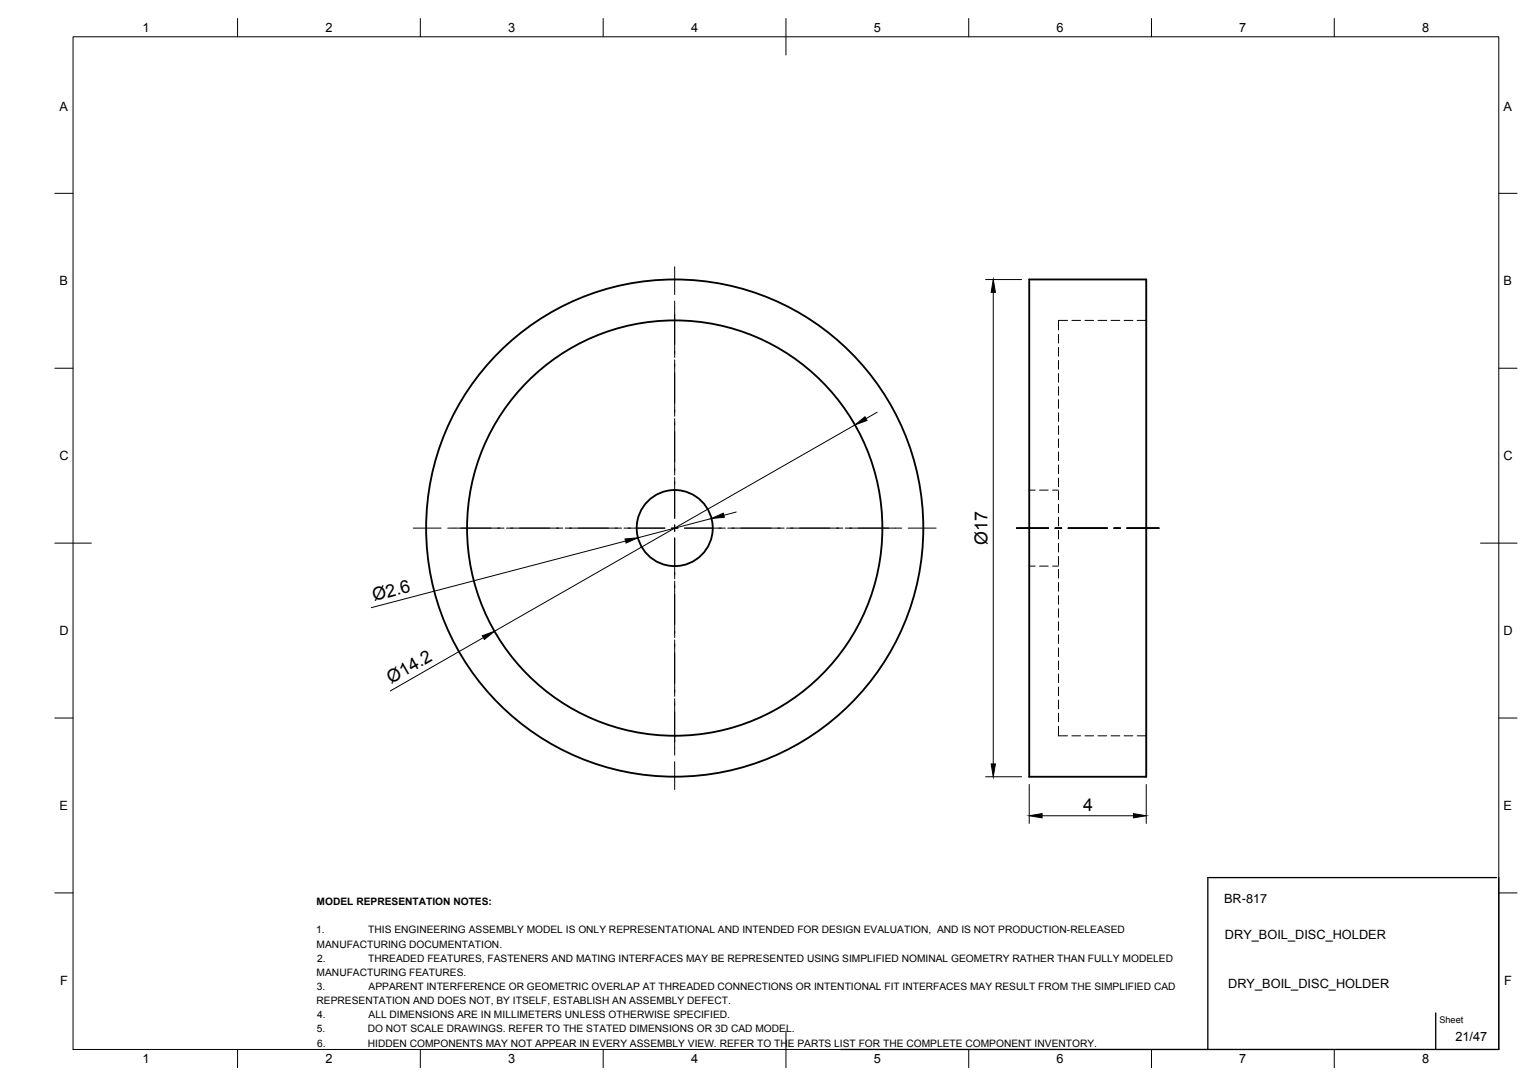
ISO-10303-21;
HEADER;
FILE_DESCRIPTION((''),'2;1');
FILE_NAME('DRY_BOIL_DISC_HOLDER.step','2026-10-01T22:07:29-07:00',(''),(''),'','','');
FILE_SCHEMA (('AUTOMOTIVE_DESIGN { 1 0 10303 214 3 1 1 }'));
ENDSEC;
DATA;
#10=MECHANICAL_DESIGN_GEOMETRIC_PRESENTATION_REPRESENTATION('',(#555),#15484);
#485=SHAPE_REPRESENTATION_RELATIONSHIP('SRR','None',#15634,#520) ;
#520=ADVANCED_BREP_SHAPE_REPRESENTATION('',(#596),#15458) ;
#555=STYLED_ITEM('',(#15834),#596) ;
#596=MANIFOLD_SOLID_BREP('DRY_BOIL_DISC_HOLDER',#8266) ;
#677=CYLINDRICAL_SURFACE('',#8977,0.13) ;
#678=CYLINDRICAL_SURFACE('',#8980,0.71) ;
#679=CYLINDRICAL_SURFACE('',#8985,0.85) ;
#863=FACE_BOUND('',#2079,.T.) ;
#864=FACE_BOUND('',#2082,.T.) ;
#865=FACE_BOUND('',#2084,.T.) ;
#997=CIRCLE('',#8978,0.13) ;
#998=CIRCLE('',#8979,0.13) ;
#999=CIRCLE('',#8981,0.71) ;
#1000=CIRCLE('',#8982,0.71) ;
#1001=CIRCLE('',#8984,0.85) ;
#1002=CIRCLE('',#8986,0.85) ;
#1523=FACE_OUTER_BOUND('',#2076,.T.) ;
#1524=FACE_OUTER_BOUND('',#2077,.T.) ;
#1525=FACE_OUTER_BOUND('',#2078,.T.) ;
#1526=FACE_OUTER_BOUND('',#2080,.T.) ;
#1527=FACE_OUTER_BOUND('',#2081,.T.) ;
#1528=FACE_OUTER_BOUND('',#2083,.T.) ;
#2076=EDGE_LOOP('',(#5913,#5914,#5915,#5916)) ;
#2077=EDGE_LOOP('',(#5917,#5918,#5919,#5920)) ;
#2078=EDGE_LOOP('',(#5921)) ;
#2079=EDGE_LOOP('',(#5922)) ;
#2080=EDGE_LOOP('',(#5923,#5924,#5925,#5926)) ;
#2081=EDGE_LOOP('',(#5927)) ;
#2082=EDGE_LOOP('',(#5928)) ;
#2083=EDGE_LOOP('',(#5929)) ;
#2084=EDGE_LOOP('',(#5930)) ;
#2644=LINE('',#13647,#3118) ;
#2645=LINE('',#13653,#3119) ;
#2646=LINE('',#13660,#3120) ;
#3118=VECTOR('',#10723,0.13) ;
#3119=VECTOR('',#10730,0.71) ;
#3120=VECTOR('',#10739,0.85) ;
#3603=VERTEX_POINT('',#13644) ;
#3604=VERTEX_POINT('',#13646) ;
#3605=VERTEX_POINT('',#13650) ;
#3606=VERTEX_POINT('',#13652) ;
#3607=VERTEX_POINT('',#13656) ;
#3608=VERTEX_POINT('',#13659) ;
#4461=EDGE_CURVE('',#3603,#3603,#997,.T.) ;
#4462=EDGE_CURVE('',#3603,#3604,#2644,.T.) ;
#4463=EDGE_CURVE('',#3604,#3604,#998,.T.) ;
#4464=EDGE_CURVE('',#3605,#3605,#999,.T.) ;
#4465=EDGE_CURVE('',#3605,#3606,#2645,.T.) ;
#4466=EDGE_CURVE('',#3606,#3606,#1000,.T.) ;
#4467=EDGE_CURVE('',#3607,#3607,#1001,.T.) ;
#4468=EDGE_CURVE('',#3607,#3608,#2646,.T.) ;
#4469=EDGE_CURVE('',#3608,#3608,#1002,.T.) ;
#5913=ORIENTED_EDGE('',*,*,#4461,.F.) ;
#5914=ORIENTED_EDGE('',*,*,#4462,.T.) ;
#5915=ORIENTED_EDGE('',*,*,#4463,.F.) ;
#5916=ORIENTED_EDGE('',*,*,#4462,.F.) ;
#5917=ORIENTED_EDGE('',*,*,#4464,.F.) ;
#5918=ORIENTED_EDGE('',*,*,#4465,.T.) ;
#5919=ORIENTED_EDGE('',*,*,#4466,.F.) ;
#5920=ORIENTED_EDGE('',*,*,#4465,.F.) ;
#5921=ORIENTED_EDGE('',*,*,#4467,.T.) ;
#5922=ORIENTED_EDGE('',*,*,#4466,.T.) ;
#5923=ORIENTED_EDGE('',*,*,#4467,.F.) ;
#5924=ORIENTED_EDGE('',*,*,#4468,.T.) ;
#5925=ORIENTED_EDGE('',*,*,#4469,.F.) ;
#5926=ORIENTED_EDGE('',*,*,#4468,.F.) ;
#5927=ORIENTED_EDGE('',*,*,#4469,.T.) ;
#5928=ORIENTED_EDGE('',*,*,#4461,.T.) ;
#5929=ORIENTED_EDGE('',*,*,#4464,.T.) ;
#5930=ORIENTED_EDGE('',*,*,#4463,.T.) ;
#7638=PLANE('',#8983) ;
#7639=PLANE('',#8987) ;
#7640=PLANE('',#8988) ;
#7910=ADVANCED_FACE('',(#1523),#677,.F.) ;
#7911=ADVANCED_FACE('',(#1524),#678,.F.) ;
#7912=ADVANCED_FACE('',(#1525,#863),#7638,.T.) ;
#7913=ADVANCED_FACE('',(#1526),#679,.T.) ;
#7914=ADVANCED_FACE('',(#1527,#864),#7639,.T.) ;
#7915=ADVANCED_FACE('',(#1528,#865),#7640,.T.) ;
#8266=CLOSED_SHELL('',(#7910,#7911,#7912,#7913,#7914,#7915)) ;
#8976=AXIS2_PLACEMENT_3D('',#13642,#10717,#10718) ;
#8977=AXIS2_PLACEMENT_3D('',#13643,#10719,#10720) ;
#8978=AXIS2_PLACEMENT_3D('',#13645,#10721,#10722) ;
#8979=AXIS2_PLACEMENT_3D('',#13648,#10724,#10725) ;
#8980=AXIS2_PLACEMENT_3D('',#13649,#10726,#10727) ;
#8981=AXIS2_PLACEMENT_3D('',#13651,#10728,#10729) ;
#8982=AXIS2_PLACEMENT_3D('',#13654,#10731,#10732) ;
#8983=AXIS2_PLACEMENT_3D('',#13655,#10733,#10734) ;
#8984=AXIS2_PLACEMENT_3D('',#13657,#10735,#10736) ;
#8985=AXIS2_PLACEMENT_3D('',#13658,#10737,#10738) ;
#8986=AXIS2_PLACEMENT_3D('',#13661,#10740,#10741) ;
#8987=AXIS2_PLACEMENT_3D('',#13662,#10742,#10743) ;
#8988=AXIS2_PLACEMENT_3D('',#13663,#10744,#10745) ;
#10717=DIRECTION('axis',(0.,0.,1.)) ;
#10718=DIRECTION('refdir',(1.,0.,0.)) ;
#10719=DIRECTION('center_axis',(0.,0.,1.)) ;
#10720=DIRECTION('ref_axis',(1.,0.,0.)) ;
#10721=DIRECTION('center_axis',(0.,0.,1.)) ;
#10722=DIRECTION('ref_axis',(1.,0.,0.)) ;
#10723=DIRECTION('',(0.,0.,1.)) ;
#10724=DIRECTION('center_axis',(0.,0.,-1.)) ;
#10725=DIRECTION('ref_axis',(1.,0.,0.)) ;
#10726=DIRECTION('center_axis',(0.,0.,1.)) ;
#10727=DIRECTION('ref_axis',(1.,0.,0.)) ;
#10728=DIRECTION('center_axis',(0.,0.,1.)) ;
#10729=DIRECTION('ref_axis',(1.,0.,0.)) ;
#10730=DIRECTION('',(0.,0.,1.)) ;
#10731=DIRECTION('center_axis',(0.,0.,-1.)) ;
#10732=DIRECTION('ref_axis',(1.,0.,0.)) ;
#10733=DIRECTION('center_axis',(0.,0.,1.)) ;
#10734=DIRECTION('ref_axis',(1.,0.,0.)) ;
#10735=DIRECTION('center_axis',(0.,0.,1.)) ;
#10736=DIRECTION('ref_axis',(1.,0.,0.)) ;
#10737=DIRECTION('center_axis',(0.,0.,1.)) ;
#10738=DIRECTION('ref_axis',(1.,0.,0.)) ;
#10739=DIRECTION('',(0.,0.,-1.)) ;
#10740=DIRECTION('center_axis',(0.,0.,-1.)) ;
#10741=DIRECTION('ref_axis',(1.,0.,0.)) ;
#10742=DIRECTION('center_axis',(0.,0.,-1.)) ;
#10743=DIRECTION('ref_axis',(-1.,0.,0.)) ;
#10744=DIRECTION('center_axis',(0.,0.,1.)) ;
#10745=DIRECTION('ref_axis',(1.,0.,0.)) ;
#13642=CARTESIAN_POINT('',(0.,0.,0.)) ;
#13643=CARTESIAN_POINT('Origin',(0.,-1.4,1.15)) ;
#13644=CARTESIAN_POINT('',(-0.13,-1.4,1.1)) ;
#13645=CARTESIAN_POINT('Origin',(0.,-1.4,1.1)) ;
#13646=CARTESIAN_POINT('',(-0.13,-1.4,1.2)) ;
#13647=CARTESIAN_POINT('',(-0.13,-1.4,1.15)) ;
#13648=CARTESIAN_POINT('Origin',(0.,-1.4,1.2)) ;
#13649=CARTESIAN_POINT('Origin',(0.,-1.4,1.35)) ;
#13650=CARTESIAN_POINT('',(-0.71,-1.4,1.2)) ;
#13651=CARTESIAN_POINT('Origin',(0.,-1.4,1.2)) ;
#13652=CARTESIAN_POINT('',(-0.71,-1.4,1.5)) ;
#13653=CARTESIAN_POINT('',(-0.71,-1.4,1.35)) ;
#13654=CARTESIAN_POINT('Origin',(0.,-1.4,1.5)) ;
#13655=CARTESIAN_POINT('Origin',(0.,-1.4,1.5)) ;
#13656=CARTESIAN_POINT('',(-0.85,-1.4,1.5)) ;
#13657=CARTESIAN_POINT('Origin',(0.,-1.4,1.5)) ;
#13658=CARTESIAN_POINT('Origin',(0.,-1.4,1.15)) ;
#13659=CARTESIAN_POINT('',(-0.85,-1.4,1.1)) ;
#13660=CARTESIAN_POINT('',(-0.85,-1.4,1.15)) ;
#13661=CARTESIAN_POINT('Origin',(0.,-1.4,1.1)) ;
#13662=CARTESIAN_POINT('Origin',(0.,-1.4,1.1)) ;
#13663=CARTESIAN_POINT('Origin',(0.,-1.4,1.2)) ;
#15415=UNCERTAINTY_MEASURE_WITH_UNIT(LENGTH_MEASURE(0.001),#15485,
'DISTANCE_ACCURACY_VALUE',
'Maximum model space distance between geometric entities at asserted c
onnectivities') ;
#15441=UNCERTAINTY_MEASURE_WITH_UNIT(LENGTH_MEASURE(0.001),#15485,
'DISTANCE_ACCURACY_VALUE',
'Maximum model space distance between geometric entities at asserted c
onnectivities') ;
#15458=(
GEOMETRIC_REPRESENTATION_CONTEXT(3)
GLOBAL_UNCERTAINTY_ASSIGNED_CONTEXT((#15415))
GLOBAL_UNIT_ASSIGNED_CONTEXT((#15485,#15487,#15488))
REPRESENTATION_CONTEXT('','3D')
) ;
#15484=(
GEOMETRIC_REPRESENTATION_CONTEXT(3)
GLOBAL_UNCERTAINTY_ASSIGNED_CONTEXT((#15441))
GLOBAL_UNIT_ASSIGNED_CONTEXT((#15485,#15487,#15488))
REPRESENTATION_CONTEXT('','3D')
) ;
#15485=(
LENGTH_UNIT()
NAMED_UNIT(*)
SI_UNIT(.CENTI.,.METRE.)
) ;
#15487=(
NAMED_UNIT(*)
PLANE_ANGLE_UNIT()
SI_UNIT($,.RADIAN.)
) ;
#15488=(
NAMED_UNIT(*)
SI_UNIT($,.STERADIAN.)
SOLID_ANGLE_UNIT()
) ;
#15505=SHAPE_DEFINITION_REPRESENTATION(#15553,#15634) ;
#15553=PRODUCT_DEFINITION_SHAPE('',$,#15677) ;
#15634=SHAPE_REPRESENTATION('',(#8976),#15458) ;
#15660=PRODUCT_DEFINITION_CONTEXT('part definition',#15788,'design') ;
#15677=PRODUCT_DEFINITION('DRY_BOIL_DISC_HOLDER',
'DRY_BOIL_DISC_HOLDER',#15719,#15660) ;
#15719=PRODUCT_DEFINITION_FORMATION('',$,#15806) ;
#15788=APPLICATION_CONTEXT(
'Core Data for Automotive Mechanical Design Process') ;
#15789=PRODUCT_CONTEXT('part definition',#15788,'mechanical') ;
#15806=PRODUCT('DRY_BOIL_DISC_HOLDER','DRY_BOIL_DISC_HOLDER',$,(#15789)) ;
#15834=PRESENTATION_STYLE_ASSIGNMENT((#15846)) ;
#15846=SURFACE_STYLE_USAGE(.BOTH.,#15858) ;
#15858=SURFACE_SIDE_STYLE('',(#15870)) ;
#15870=SURFACE_STYLE_FILL_AREA(#15882) ;
#15882=FILL_AREA_STYLE('Brass - Polished',(#15894)) ;
#15894=FILL_AREA_STYLE_COLOUR('Brass - Polished',#15906) ;
#15906=COLOUR_RGB('Brass - Polished', 0.08235294, 0.09019608, 0.10196078) ;
ENDSEC;
END-ISO-10303-21;
